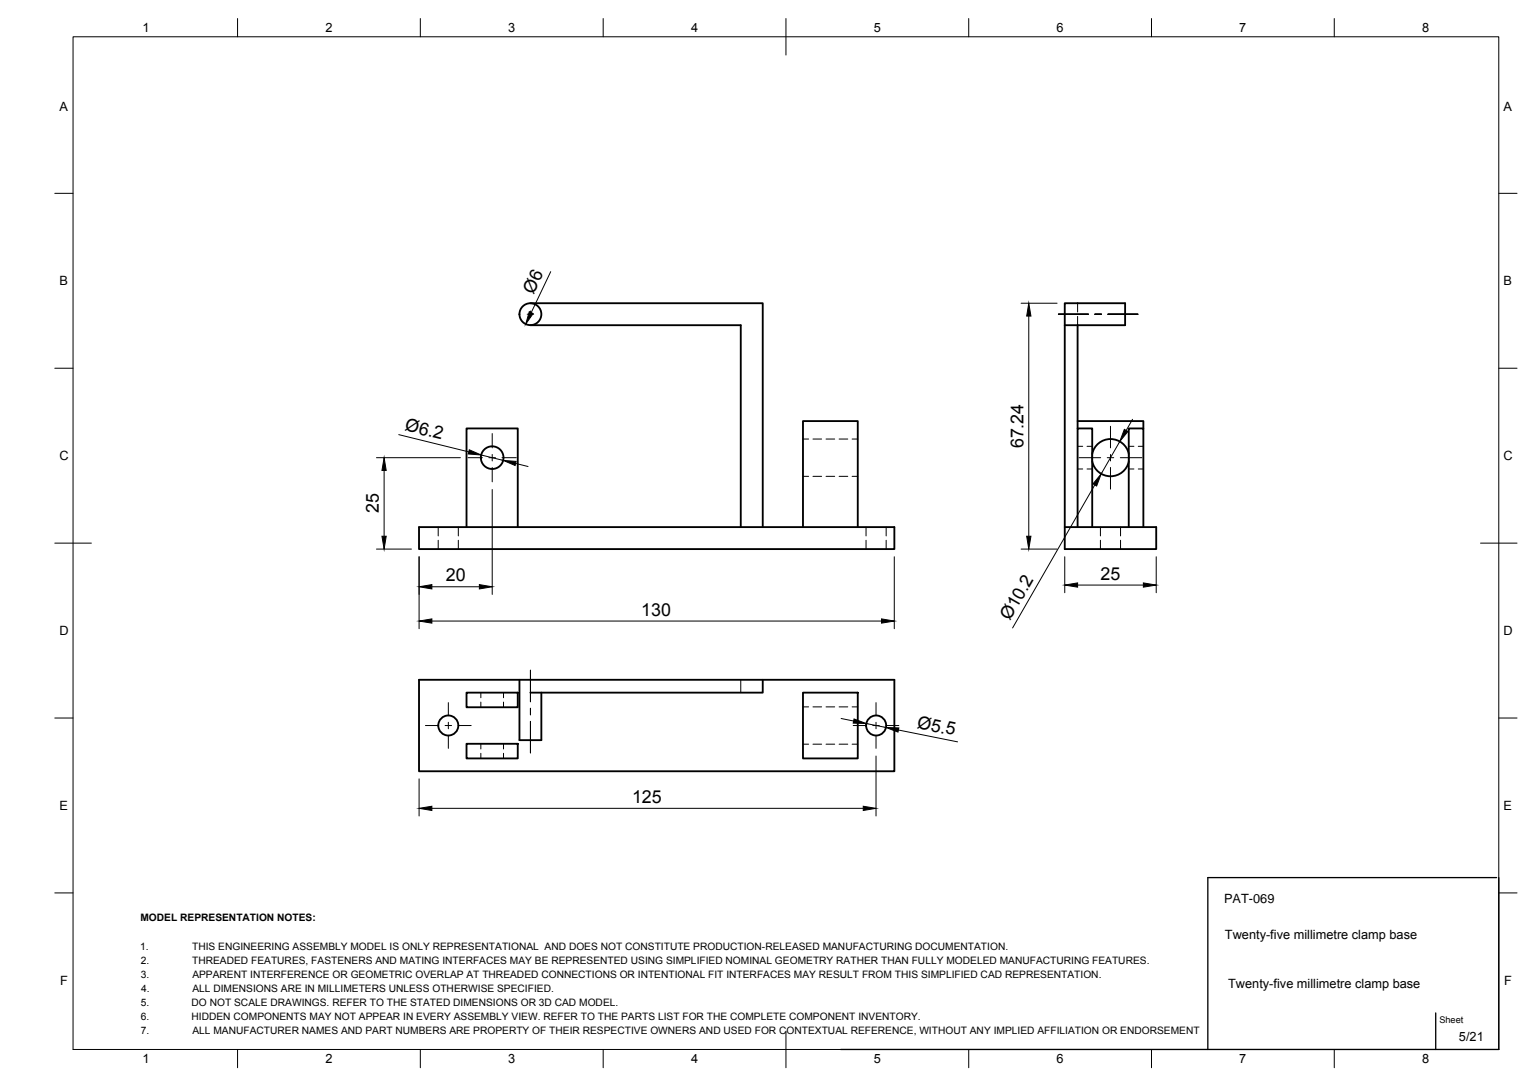
ISO-10303-21;
HEADER;
/* Generated by software containing ST-Developer
 * from STEP Tools, Inc. (www.steptools.com) 
 */

FILE_DESCRIPTION(
/* description */ ('Located fixture plate with toggle clamp'),
/* implementation_level */ '2;1');

FILE_NAME(
/* name */ 'Twenty-five millimetre clamp base.step',
/* time_stamp */ '2026-10-27T21:36:12-07:00',
/* author */ (''),
/* organization */ (''),
/* preprocessor_version */ 'ST-DEVELOPER v20.2',
/* originating_system */ 'Autodesk Translation Framework v15.17.0.0',
/* authorisation */ '');

FILE_SCHEMA (('AUTOMOTIVE_DESIGN { 1 0 10303 214 3 1 1 }'));
ENDSEC;

DATA;
#10=MECHANICAL_DESIGN_GEOMETRIC_PRESENTATION_REPRESENTATION('',(#321),#9285);
#273=SHAPE_REPRESENTATION_RELATIONSHIP('SRR','None',#9396,#297);
#297=ADVANCED_BREP_SHAPE_REPRESENTATION('',(#345),#9258);
#321=STYLED_ITEM('',(#9591),#345);
#345=MANIFOLD_SOLID_BREP('Body1',#5169);
#366=FACE_BOUND('',#977,.T.);
#367=FACE_BOUND('',#978,.T.);
#368=FACE_BOUND('',#979,.T.);
#369=FACE_BOUND('',#980,.T.);
#370=FACE_BOUND('',#981,.T.);
#371=FACE_BOUND('',#987,.T.);
#372=FACE_BOUND('',#989,.T.);
#373=FACE_BOUND('',#995,.T.);
#374=FACE_BOUND('',#1000,.T.);
#375=FACE_BOUND('',#1002,.T.);
#376=FACE_BOUND('',#1007,.T.);
#377=FACE_BOUND('',#1012,.T.);
#378=FACE_BOUND('',#1013,.T.);
#486=PLANE('',#5469);
#487=PLANE('',#5470);
#488=PLANE('',#5471);
#489=PLANE('',#5472);
#490=PLANE('',#5473);
#491=PLANE('',#5474);
#492=PLANE('',#5475);
#493=PLANE('',#5476);
#494=PLANE('',#5486);
#495=PLANE('',#5487);
#496=PLANE('',#5488);
#497=PLANE('',#5489);
#498=PLANE('',#5490);
#499=PLANE('',#5497);
#500=PLANE('',#5498);
#501=PLANE('',#5499);
#502=PLANE('',#5500);
#503=PLANE('',#5501);
#504=PLANE('',#5502);
#505=PLANE('',#5503);
#506=PLANE('',#5504);
#507=PLANE('',#5505);
#508=PLANE('',#5506);
#509=PLANE('',#5507);
#510=PLANE('',#5508);
#511=PLANE('',#5509);
#512=PLANE('',#5510);
#673=FACE_OUTER_BOUND('',#968,.T.);
#674=FACE_OUTER_BOUND('',#969,.T.);
#675=FACE_OUTER_BOUND('',#970,.T.);
#676=FACE_OUTER_BOUND('',#971,.T.);
#677=FACE_OUTER_BOUND('',#972,.T.);
#678=FACE_OUTER_BOUND('',#973,.T.);
#679=FACE_OUTER_BOUND('',#974,.T.);
#680=FACE_OUTER_BOUND('',#975,.T.);
#681=FACE_OUTER_BOUND('',#976,.T.);
#682=FACE_OUTER_BOUND('',#982,.T.);
#683=FACE_OUTER_BOUND('',#983,.T.);
#684=FACE_OUTER_BOUND('',#984,.T.);
#685=FACE_OUTER_BOUND('',#985,.T.);
#686=FACE_OUTER_BOUND('',#986,.T.);
#687=FACE_OUTER_BOUND('',#988,.T.);
#688=FACE_OUTER_BOUND('',#990,.T.);
#689=FACE_OUTER_BOUND('',#991,.T.);
#690=FACE_OUTER_BOUND('',#992,.T.);
#691=FACE_OUTER_BOUND('',#993,.T.);
#692=FACE_OUTER_BOUND('',#994,.T.);
#693=FACE_OUTER_BOUND('',#996,.T.);
#694=FACE_OUTER_BOUND('',#997,.T.);
#695=FACE_OUTER_BOUND('',#998,.T.);
#696=FACE_OUTER_BOUND('',#999,.T.);
#697=FACE_OUTER_BOUND('',#1001,.T.);
#698=FACE_OUTER_BOUND('',#1003,.T.);
#699=FACE_OUTER_BOUND('',#1004,.T.);
#700=FACE_OUTER_BOUND('',#1005,.T.);
#701=FACE_OUTER_BOUND('',#1006,.T.);
#702=FACE_OUTER_BOUND('',#1008,.T.);
#703=FACE_OUTER_BOUND('',#1009,.T.);
#704=FACE_OUTER_BOUND('',#1010,.T.);
#705=FACE_OUTER_BOUND('',#1011,.T.);
#968=EDGE_LOOP('',(#3484,#3485,#3486,#3487,#3488,#3489,#3490,#3491));
#969=EDGE_LOOP('',(#3492));
#970=EDGE_LOOP('',(#3493,#3494,#3495,#3496,#3497,#3498,#3499,#3500,#3501,
#3502,#3503));
#971=EDGE_LOOP('',(#3504,#3505,#3506,#3507));
#972=EDGE_LOOP('',(#3508,#3509,#3510,#3511));
#973=EDGE_LOOP('',(#3512,#3513,#3514,#3515));
#974=EDGE_LOOP('',(#3516,#3517,#3518,#3519));
#975=EDGE_LOOP('',(#3520,#3521,#3522,#3523,#3524,#3525));
#976=EDGE_LOOP('',(#3526,#3527,#3528,#3529,#3530,#3531,#3532,#3533));
#977=EDGE_LOOP('',(#3534,#3535,#3536,#3537));
#978=EDGE_LOOP('',(#3538,#3539,#3540,#3541));
#979=EDGE_LOOP('',(#3542,#3543,#3544,#3545));
#980=EDGE_LOOP('',(#3546));
#981=EDGE_LOOP('',(#3547));
#982=EDGE_LOOP('',(#3548,#3549,#3550,#3551));
#983=EDGE_LOOP('',(#3552,#3553,#3554,#3555));
#984=EDGE_LOOP('',(#3556,#3557,#3558,#3559));
#985=EDGE_LOOP('',(#3560,#3561,#3562,#3563));
#986=EDGE_LOOP('',(#3564,#3565,#3566,#3567));
#987=EDGE_LOOP('',(#3568));
#988=EDGE_LOOP('',(#3569,#3570,#3571,#3572));
#989=EDGE_LOOP('',(#3573));
#990=EDGE_LOOP('',(#3574,#3575,#3576,#3577));
#991=EDGE_LOOP('',(#3578,#3579,#3580,#3581));
#992=EDGE_LOOP('',(#3582,#3583,#3584,#3585));
#993=EDGE_LOOP('',(#3586,#3587,#3588,#3589));
#994=EDGE_LOOP('',(#3590,#3591,#3592,#3593));
#995=EDGE_LOOP('',(#3594));
#996=EDGE_LOOP('',(#3595,#3596,#3597,#3598));
#997=EDGE_LOOP('',(#3599,#3600,#3601,#3602));
#998=EDGE_LOOP('',(#3603,#3604,#3605,#3606));
#999=EDGE_LOOP('',(#3607,#3608,#3609,#3610));
#1000=EDGE_LOOP('',(#3611));
#1001=EDGE_LOOP('',(#3612,#3613,#3614,#3615));
#1002=EDGE_LOOP('',(#3616));
#1003=EDGE_LOOP('',(#3617,#3618,#3619,#3620));
#1004=EDGE_LOOP('',(#3621,#3622,#3623,#3624));
#1005=EDGE_LOOP('',(#3625,#3626,#3627,#3628));
#1006=EDGE_LOOP('',(#3629,#3630,#3631,#3632));
#1007=EDGE_LOOP('',(#3633));
#1008=EDGE_LOOP('',(#3634,#3635,#3636,#3637));
#1009=EDGE_LOOP('',(#3638,#3639,#3640,#3641));
#1010=EDGE_LOOP('',(#3642,#3643,#3644,#3645));
#1011=EDGE_LOOP('',(#3646,#3647,#3648,#3649));
#1012=EDGE_LOOP('',(#3650));
#1013=EDGE_LOOP('',(#3651));
#1383=CIRCLE('',#5465,0.3);
#1384=CIRCLE('',#5466,0.3);
#1385=CIRCLE('',#5467,0.3);
#1386=CIRCLE('',#5468,0.3);
#1387=CIRCLE('',#5477,0.275);
#1388=CIRCLE('',#5478,0.275);
#1389=CIRCLE('',#5480,0.275);
#1390=CIRCLE('',#5482,0.275);
#1391=CIRCLE('',#5484,0.51);
#1392=CIRCLE('',#5485,0.51);
#1393=CIRCLE('',#5492,0.31);
#1394=CIRCLE('',#5493,0.31);
#1395=CIRCLE('',#5495,0.31);
#1396=CIRCLE('',#5496,0.31);
#1581=LINE('',#7581,#1991);
#1582=LINE('',#7585,#1992);
#1583=LINE('',#7589,#1993);
#1584=LINE('',#7595,#1994);
#1585=LINE('',#7597,#1995);
#1586=LINE('',#7599,#1996);
#1587=LINE('',#7601,#1997);
#1588=LINE('',#7603,#1998);
#1589=LINE('',#7605,#1999);
#1590=LINE('',#7607,#2000);
#1591=LINE('',#7609,#2001);
#1592=LINE('',#7610,#2002);
#1593=LINE('',#7613,#2003);
#1594=LINE('',#7614,#2004);
#1595=LINE('',#7617,#2005);
#1596=LINE('',#7618,#2006);
#1597=LINE('',#7621,#2007);
#1598=LINE('',#7622,#2008);
#1599=LINE('',#7625,#2009);
#1600=LINE('',#7626,#2010);
#1601=LINE('',#7628,#2011);
#1602=LINE('',#7631,#2012);
#1603=LINE('',#7633,#2013);
#1604=LINE('',#7634,#2014);
#1605=LINE('',#7637,#2015);
#1606=LINE('',#7639,#2016);
#1607=LINE('',#7641,#2017);
#1608=LINE('',#7642,#2018);
#1609=LINE('',#7645,#2019);
#1610=LINE('',#7647,#2020);
#1611=LINE('',#7649,#2021);
#1612=LINE('',#7650,#2022);
#1613=LINE('',#7653,#2023);
#1614=LINE('',#7655,#2024);
#1615=LINE('',#7657,#2025);
#1616=LINE('',#7658,#2026);
#1617=LINE('',#7666,#2027);
#1618=LINE('',#7670,#2028);
#1619=LINE('',#7675,#2029);
#1620=LINE('',#7679,#2030);
#1621=LINE('',#7681,#2031);
#1622=LINE('',#7682,#2032);
#1623=LINE('',#7685,#2033);
#1624=LINE('',#7686,#2034);
#1625=LINE('',#7689,#2035);
#1626=LINE('',#7690,#2036);
#1627=LINE('',#7692,#2037);
#1628=LINE('',#7698,#2038);
#1629=LINE('',#7704,#2039);
#1630=LINE('',#7708,#2040);
#1631=LINE('',#7710,#2041);
#1632=LINE('',#7711,#2042);
#1633=LINE('',#7714,#2043);
#1634=LINE('',#7715,#2044);
#1635=LINE('',#7718,#2045);
#1636=LINE('',#7719,#2046);
#1637=LINE('',#7721,#2047);
#1638=LINE('',#7725,#2048);
#1639=LINE('',#7727,#2049);
#1640=LINE('',#7728,#2050);
#1641=LINE('',#7731,#2051);
#1642=LINE('',#7732,#2052);
#1643=LINE('',#7735,#2053);
#1644=LINE('',#7736,#2054);
#1645=LINE('',#7738,#2055);
#1646=LINE('',#7742,#2056);
#1647=LINE('',#7743,#2057);
#1648=LINE('',#7746,#2058);
#1649=LINE('',#7747,#2059);
#1650=LINE('',#7749,#2060);
#1991=VECTOR('',#6037,1.);
#1992=VECTOR('',#6040,1.);
#1993=VECTOR('',#6043,0.3);
#1994=VECTOR('',#6052,1.);
#1995=VECTOR('',#6053,1.);
#1996=VECTOR('',#6054,1.);
#1997=VECTOR('',#6055,1.);
#1998=VECTOR('',#6056,1.);
#1999=VECTOR('',#6057,1.);
#2000=VECTOR('',#6058,1.);
#2001=VECTOR('',#6059,1.);
#2002=VECTOR('',#6060,1.);
#2003=VECTOR('',#6063,1.);
#2004=VECTOR('',#6064,1.);
#2005=VECTOR('',#6067,1.);
#2006=VECTOR('',#6068,1.);
#2007=VECTOR('',#6071,1.);
#2008=VECTOR('',#6072,1.);
#2009=VECTOR('',#6075,1.);
#2010=VECTOR('',#6076,1.);
#2011=VECTOR('',#6079,1.);
#2012=VECTOR('',#6082,1.);
#2013=VECTOR('',#6083,1.);
#2014=VECTOR('',#6084,1.);
#2015=VECTOR('',#6085,1.);
#2016=VECTOR('',#6086,1.);
#2017=VECTOR('',#6087,1.);
#2018=VECTOR('',#6088,1.);
#2019=VECTOR('',#6089,1.);
#2020=VECTOR('',#6090,1.);
#2021=VECTOR('',#6091,1.);
#2022=VECTOR('',#6092,1.);
#2023=VECTOR('',#6093,1.);
#2024=VECTOR('',#6094,1.);
#2025=VECTOR('',#6095,1.);
#2026=VECTOR('',#6096,1.);
#2027=VECTOR('',#6105,0.275);
#2028=VECTOR('',#6110,0.275);
#2029=VECTOR('',#6115,0.51);
#2030=VECTOR('',#6120,1.);
#2031=VECTOR('',#6121,1.);
#2032=VECTOR('',#6122,1.);
#2033=VECTOR('',#6125,1.);
#2034=VECTOR('',#6126,1.);
#2035=VECTOR('',#6129,1.);
#2036=VECTOR('',#6130,1.);
#2037=VECTOR('',#6133,1.);
#2038=VECTOR('',#6140,0.31);
#2039=VECTOR('',#6147,0.31);
#2040=VECTOR('',#6152,1.);
#2041=VECTOR('',#6153,1.);
#2042=VECTOR('',#6154,1.);
#2043=VECTOR('',#6157,1.);
#2044=VECTOR('',#6158,1.);
#2045=VECTOR('',#6161,1.);
#2046=VECTOR('',#6162,1.);
#2047=VECTOR('',#6165,1.);
#2048=VECTOR('',#6170,1.);
#2049=VECTOR('',#6171,1.);
#2050=VECTOR('',#6172,1.);
#2051=VECTOR('',#6175,1.);
#2052=VECTOR('',#6176,1.);
#2053=VECTOR('',#6179,1.);
#2054=VECTOR('',#6180,1.);
#2055=VECTOR('',#6183,1.);
#2056=VECTOR('',#6188,1.);
#2057=VECTOR('',#6189,1.);
#2058=VECTOR('',#6192,1.);
#2059=VECTOR('',#6193,1.);
#2060=VECTOR('',#6196,1.);
#2401=VERTEX_POINT('',#7579);
#2402=VERTEX_POINT('',#7580);
#2403=VERTEX_POINT('',#7582);
#2404=VERTEX_POINT('',#7584);
#2405=VERTEX_POINT('',#7586);
#2406=VERTEX_POINT('',#7588);
#2407=VERTEX_POINT('',#7594);
#2408=VERTEX_POINT('',#7596);
#2409=VERTEX_POINT('',#7598);
#2410=VERTEX_POINT('',#7600);
#2411=VERTEX_POINT('',#7602);
#2412=VERTEX_POINT('',#7604);
#2413=VERTEX_POINT('',#7606);
#2414=VERTEX_POINT('',#7608);
#2415=VERTEX_POINT('',#7612);
#2416=VERTEX_POINT('',#7616);
#2417=VERTEX_POINT('',#7620);
#2418=VERTEX_POINT('',#7624);
#2419=VERTEX_POINT('',#7630);
#2420=VERTEX_POINT('',#7632);
#2421=VERTEX_POINT('',#7635);
#2422=VERTEX_POINT('',#7636);
#2423=VERTEX_POINT('',#7638);
#2424=VERTEX_POINT('',#7640);
#2425=VERTEX_POINT('',#7643);
#2426=VERTEX_POINT('',#7644);
#2427=VERTEX_POINT('',#7646);
#2428=VERTEX_POINT('',#7648);
#2429=VERTEX_POINT('',#7651);
#2430=VERTEX_POINT('',#7652);
#2431=VERTEX_POINT('',#7654);
#2432=VERTEX_POINT('',#7656);
#2433=VERTEX_POINT('',#7659);
#2434=VERTEX_POINT('',#7661);
#2435=VERTEX_POINT('',#7664);
#2436=VERTEX_POINT('',#7668);
#2437=VERTEX_POINT('',#7672);
#2438=VERTEX_POINT('',#7674);
#2439=VERTEX_POINT('',#7678);
#2440=VERTEX_POINT('',#7680);
#2441=VERTEX_POINT('',#7684);
#2442=VERTEX_POINT('',#7688);
#2443=VERTEX_POINT('',#7695);
#2444=VERTEX_POINT('',#7697);
#2445=VERTEX_POINT('',#7701);
#2446=VERTEX_POINT('',#7703);
#2447=VERTEX_POINT('',#7707);
#2448=VERTEX_POINT('',#7709);
#2449=VERTEX_POINT('',#7713);
#2450=VERTEX_POINT('',#7717);
#2451=VERTEX_POINT('',#7724);
#2452=VERTEX_POINT('',#7726);
#2453=VERTEX_POINT('',#7730);
#2454=VERTEX_POINT('',#7734);
#2455=VERTEX_POINT('',#7741);
#2456=VERTEX_POINT('',#7745);
#2830=EDGE_CURVE('',#2401,#2402,#1581,.T.);
#2831=EDGE_CURVE('',#2403,#2401,#1383,.T.);
#2832=EDGE_CURVE('',#2403,#2404,#1582,.T.);
#2833=EDGE_CURVE('',#2405,#2404,#1384,.T.);
#2834=EDGE_CURVE('',#2405,#2406,#1583,.T.);
#2835=EDGE_CURVE('',#2406,#2406,#1385,.T.);
#2836=EDGE_CURVE('',#2402,#2405,#1386,.T.);
#2837=EDGE_CURVE('',#2404,#2407,#1584,.T.);
#2838=EDGE_CURVE('',#2407,#2408,#1585,.T.);
#2839=EDGE_CURVE('',#2409,#2408,#1586,.T.);
#2840=EDGE_CURVE('',#2410,#2409,#1587,.T.);
#2841=EDGE_CURVE('',#2410,#2411,#1588,.T.);
#2842=EDGE_CURVE('',#2411,#2412,#1589,.T.);
#2843=EDGE_CURVE('',#2413,#2412,#1590,.T.);
#2844=EDGE_CURVE('',#2413,#2414,#1591,.T.);
#2845=EDGE_CURVE('',#2414,#2402,#1592,.T.);
#2846=EDGE_CURVE('',#2415,#2414,#1593,.T.);
#2847=EDGE_CURVE('',#2401,#2415,#1594,.T.);
#2848=EDGE_CURVE('',#2416,#2403,#1595,.T.);
#2849=EDGE_CURVE('',#2416,#2407,#1596,.T.);
#2850=EDGE_CURVE('',#2417,#2416,#1597,.T.);
#2851=EDGE_CURVE('',#2408,#2417,#1598,.T.);
#2852=EDGE_CURVE('',#2418,#2413,#1599,.T.);
#2853=EDGE_CURVE('',#2415,#2418,#1600,.T.);
#2854=EDGE_CURVE('',#2417,#2418,#1601,.T.);
#2855=EDGE_CURVE('',#2412,#2419,#1602,.T.);
#2856=EDGE_CURVE('',#2419,#2420,#1603,.T.);
#2857=EDGE_CURVE('',#2420,#2409,#1604,.T.);
#2858=EDGE_CURVE('',#2421,#2422,#1605,.T.);
#2859=EDGE_CURVE('',#2422,#2423,#1606,.T.);
#2860=EDGE_CURVE('',#2423,#2424,#1607,.T.);
#2861=EDGE_CURVE('',#2424,#2421,#1608,.T.);
#2862=EDGE_CURVE('',#2425,#2426,#1609,.T.);
#2863=EDGE_CURVE('',#2426,#2427,#1610,.T.);
#2864=EDGE_CURVE('',#2427,#2428,#1611,.T.);
#2865=EDGE_CURVE('',#2428,#2425,#1612,.T.);
#2866=EDGE_CURVE('',#2429,#2430,#1613,.T.);
#2867=EDGE_CURVE('',#2430,#2431,#1614,.T.);
#2868=EDGE_CURVE('',#2431,#2432,#1615,.T.);
#2869=EDGE_CURVE('',#2432,#2429,#1616,.T.);
#2870=EDGE_CURVE('',#2433,#2433,#1387,.T.);
#2871=EDGE_CURVE('',#2434,#2434,#1388,.T.);
#2872=EDGE_CURVE('',#2435,#2435,#1389,.T.);
#2873=EDGE_CURVE('',#2435,#2434,#1617,.T.);
#2874=EDGE_CURVE('',#2436,#2436,#1390,.T.);
#2875=EDGE_CURVE('',#2436,#2433,#1618,.T.);
#2876=EDGE_CURVE('',#2437,#2437,#1391,.T.);
#2877=EDGE_CURVE('',#2437,#2438,#1619,.T.);
#2878=EDGE_CURVE('',#2438,#2438,#1392,.T.);
#2879=EDGE_CURVE('',#2430,#2439,#1620,.T.);
#2880=EDGE_CURVE('',#2439,#2440,#1621,.T.);
#2881=EDGE_CURVE('',#2440,#2431,#1622,.T.);
#2882=EDGE_CURVE('',#2441,#2429,#1623,.T.);
#2883=EDGE_CURVE('',#2439,#2441,#1624,.T.);
#2884=EDGE_CURVE('',#2440,#2442,#1625,.T.);
#2885=EDGE_CURVE('',#2432,#2442,#1626,.T.);
#2886=EDGE_CURVE('',#2442,#2441,#1627,.T.);
#2887=EDGE_CURVE('',#2443,#2443,#1393,.T.);
#2888=EDGE_CURVE('',#2443,#2444,#1628,.T.);
#2889=EDGE_CURVE('',#2444,#2444,#1394,.T.);
#2890=EDGE_CURVE('',#2445,#2445,#1395,.T.);
#2891=EDGE_CURVE('',#2445,#2446,#1629,.T.);
#2892=EDGE_CURVE('',#2446,#2446,#1396,.T.);
#2893=EDGE_CURVE('',#2426,#2447,#1630,.T.);
#2894=EDGE_CURVE('',#2447,#2448,#1631,.T.);
#2895=EDGE_CURVE('',#2448,#2427,#1632,.T.);
#2896=EDGE_CURVE('',#2449,#2425,#1633,.T.);
#2897=EDGE_CURVE('',#2447,#2449,#1634,.T.);
#2898=EDGE_CURVE('',#2448,#2450,#1635,.T.);
#2899=EDGE_CURVE('',#2428,#2450,#1636,.T.);
#2900=EDGE_CURVE('',#2450,#2449,#1637,.T.);
#2901=EDGE_CURVE('',#2422,#2451,#1638,.T.);
#2902=EDGE_CURVE('',#2451,#2452,#1639,.T.);
#2903=EDGE_CURVE('',#2452,#2423,#1640,.T.);
#2904=EDGE_CURVE('',#2453,#2421,#1641,.T.);
#2905=EDGE_CURVE('',#2451,#2453,#1642,.T.);
#2906=EDGE_CURVE('',#2452,#2454,#1643,.T.);
#2907=EDGE_CURVE('',#2424,#2454,#1644,.T.);
#2908=EDGE_CURVE('',#2454,#2453,#1645,.T.);
#2909=EDGE_CURVE('',#2455,#2410,#1646,.T.);
#2910=EDGE_CURVE('',#2455,#2420,#1647,.T.);
#2911=EDGE_CURVE('',#2456,#2455,#1648,.T.);
#2912=EDGE_CURVE('',#2456,#2419,#1649,.T.);
#2913=EDGE_CURVE('',#2411,#2456,#1650,.T.);
#3484=ORIENTED_EDGE('',*,*,#2830,.F.);
#3485=ORIENTED_EDGE('',*,*,#2831,.F.);
#3486=ORIENTED_EDGE('',*,*,#2832,.T.);
#3487=ORIENTED_EDGE('',*,*,#2833,.F.);
#3488=ORIENTED_EDGE('',*,*,#2834,.T.);
#3489=ORIENTED_EDGE('',*,*,#2835,.T.);
#3490=ORIENTED_EDGE('',*,*,#2834,.F.);
#3491=ORIENTED_EDGE('',*,*,#2836,.F.);
#3492=ORIENTED_EDGE('',*,*,#2835,.F.);
#3493=ORIENTED_EDGE('',*,*,#2837,.T.);
#3494=ORIENTED_EDGE('',*,*,#2838,.T.);
#3495=ORIENTED_EDGE('',*,*,#2839,.F.);
#3496=ORIENTED_EDGE('',*,*,#2840,.F.);
#3497=ORIENTED_EDGE('',*,*,#2841,.T.);
#3498=ORIENTED_EDGE('',*,*,#2842,.T.);
#3499=ORIENTED_EDGE('',*,*,#2843,.F.);
#3500=ORIENTED_EDGE('',*,*,#2844,.T.);
#3501=ORIENTED_EDGE('',*,*,#2845,.T.);
#3502=ORIENTED_EDGE('',*,*,#2836,.T.);
#3503=ORIENTED_EDGE('',*,*,#2833,.T.);
#3504=ORIENTED_EDGE('',*,*,#2846,.F.);
#3505=ORIENTED_EDGE('',*,*,#2847,.F.);
#3506=ORIENTED_EDGE('',*,*,#2830,.T.);
#3507=ORIENTED_EDGE('',*,*,#2845,.F.);
#3508=ORIENTED_EDGE('',*,*,#2848,.F.);
#3509=ORIENTED_EDGE('',*,*,#2849,.T.);
#3510=ORIENTED_EDGE('',*,*,#2837,.F.);
#3511=ORIENTED_EDGE('',*,*,#2832,.F.);
#3512=ORIENTED_EDGE('',*,*,#2850,.F.);
#3513=ORIENTED_EDGE('',*,*,#2851,.F.);
#3514=ORIENTED_EDGE('',*,*,#2838,.F.);
#3515=ORIENTED_EDGE('',*,*,#2849,.F.);
#3516=ORIENTED_EDGE('',*,*,#2846,.T.);
#3517=ORIENTED_EDGE('',*,*,#2844,.F.);
#3518=ORIENTED_EDGE('',*,*,#2852,.F.);
#3519=ORIENTED_EDGE('',*,*,#2853,.F.);
#3520=ORIENTED_EDGE('',*,*,#2831,.T.);
#3521=ORIENTED_EDGE('',*,*,#2847,.T.);
#3522=ORIENTED_EDGE('',*,*,#2853,.T.);
#3523=ORIENTED_EDGE('',*,*,#2854,.F.);
#3524=ORIENTED_EDGE('',*,*,#2850,.T.);
#3525=ORIENTED_EDGE('',*,*,#2848,.T.);
#3526=ORIENTED_EDGE('',*,*,#2851,.T.);
#3527=ORIENTED_EDGE('',*,*,#2854,.T.);
#3528=ORIENTED_EDGE('',*,*,#2852,.T.);
#3529=ORIENTED_EDGE('',*,*,#2843,.T.);
#3530=ORIENTED_EDGE('',*,*,#2855,.T.);
#3531=ORIENTED_EDGE('',*,*,#2856,.T.);
#3532=ORIENTED_EDGE('',*,*,#2857,.T.);
#3533=ORIENTED_EDGE('',*,*,#2839,.T.);
#3534=ORIENTED_EDGE('',*,*,#2858,.T.);
#3535=ORIENTED_EDGE('',*,*,#2859,.T.);
#3536=ORIENTED_EDGE('',*,*,#2860,.T.);
#3537=ORIENTED_EDGE('',*,*,#2861,.T.);
#3538=ORIENTED_EDGE('',*,*,#2862,.T.);
#3539=ORIENTED_EDGE('',*,*,#2863,.T.);
#3540=ORIENTED_EDGE('',*,*,#2864,.T.);
#3541=ORIENTED_EDGE('',*,*,#2865,.T.);
#3542=ORIENTED_EDGE('',*,*,#2866,.T.);
#3543=ORIENTED_EDGE('',*,*,#2867,.T.);
#3544=ORIENTED_EDGE('',*,*,#2868,.T.);
#3545=ORIENTED_EDGE('',*,*,#2869,.T.);
#3546=ORIENTED_EDGE('',*,*,#2870,.T.);
#3547=ORIENTED_EDGE('',*,*,#2871,.T.);
#3548=ORIENTED_EDGE('',*,*,#2872,.F.);
#3549=ORIENTED_EDGE('',*,*,#2873,.T.);
#3550=ORIENTED_EDGE('',*,*,#2871,.F.);
#3551=ORIENTED_EDGE('',*,*,#2873,.F.);
#3552=ORIENTED_EDGE('',*,*,#2874,.F.);
#3553=ORIENTED_EDGE('',*,*,#2875,.T.);
#3554=ORIENTED_EDGE('',*,*,#2870,.F.);
#3555=ORIENTED_EDGE('',*,*,#2875,.F.);
#3556=ORIENTED_EDGE('',*,*,#2876,.F.);
#3557=ORIENTED_EDGE('',*,*,#2877,.T.);
#3558=ORIENTED_EDGE('',*,*,#2878,.F.);
#3559=ORIENTED_EDGE('',*,*,#2877,.F.);
#3560=ORIENTED_EDGE('',*,*,#2867,.F.);
#3561=ORIENTED_EDGE('',*,*,#2879,.T.);
#3562=ORIENTED_EDGE('',*,*,#2880,.T.);
#3563=ORIENTED_EDGE('',*,*,#2881,.T.);
#3564=ORIENTED_EDGE('',*,*,#2866,.F.);
#3565=ORIENTED_EDGE('',*,*,#2882,.F.);
#3566=ORIENTED_EDGE('',*,*,#2883,.F.);
#3567=ORIENTED_EDGE('',*,*,#2879,.F.);
#3568=ORIENTED_EDGE('',*,*,#2878,.T.);
#3569=ORIENTED_EDGE('',*,*,#2868,.F.);
#3570=ORIENTED_EDGE('',*,*,#2881,.F.);
#3571=ORIENTED_EDGE('',*,*,#2884,.T.);
#3572=ORIENTED_EDGE('',*,*,#2885,.F.);
#3573=ORIENTED_EDGE('',*,*,#2876,.T.);
#3574=ORIENTED_EDGE('',*,*,#2880,.F.);
#3575=ORIENTED_EDGE('',*,*,#2883,.T.);
#3576=ORIENTED_EDGE('',*,*,#2886,.F.);
#3577=ORIENTED_EDGE('',*,*,#2884,.F.);
#3578=ORIENTED_EDGE('',*,*,#2869,.F.);
#3579=ORIENTED_EDGE('',*,*,#2885,.T.);
#3580=ORIENTED_EDGE('',*,*,#2886,.T.);
#3581=ORIENTED_EDGE('',*,*,#2882,.T.);
#3582=ORIENTED_EDGE('',*,*,#2887,.F.);
#3583=ORIENTED_EDGE('',*,*,#2888,.T.);
#3584=ORIENTED_EDGE('',*,*,#2889,.F.);
#3585=ORIENTED_EDGE('',*,*,#2888,.F.);
#3586=ORIENTED_EDGE('',*,*,#2890,.F.);
#3587=ORIENTED_EDGE('',*,*,#2891,.T.);
#3588=ORIENTED_EDGE('',*,*,#2892,.F.);
#3589=ORIENTED_EDGE('',*,*,#2891,.F.);
#3590=ORIENTED_EDGE('',*,*,#2863,.F.);
#3591=ORIENTED_EDGE('',*,*,#2893,.T.);
#3592=ORIENTED_EDGE('',*,*,#2894,.T.);
#3593=ORIENTED_EDGE('',*,*,#2895,.T.);
#3594=ORIENTED_EDGE('',*,*,#2890,.T.);
#3595=ORIENTED_EDGE('',*,*,#2862,.F.);
#3596=ORIENTED_EDGE('',*,*,#2896,.F.);
#3597=ORIENTED_EDGE('',*,*,#2897,.F.);
#3598=ORIENTED_EDGE('',*,*,#2893,.F.);
#3599=ORIENTED_EDGE('',*,*,#2864,.F.);
#3600=ORIENTED_EDGE('',*,*,#2895,.F.);
#3601=ORIENTED_EDGE('',*,*,#2898,.T.);
#3602=ORIENTED_EDGE('',*,*,#2899,.F.);
#3603=ORIENTED_EDGE('',*,*,#2894,.F.);
#3604=ORIENTED_EDGE('',*,*,#2897,.T.);
#3605=ORIENTED_EDGE('',*,*,#2900,.F.);
#3606=ORIENTED_EDGE('',*,*,#2898,.F.);
#3607=ORIENTED_EDGE('',*,*,#2865,.F.);
#3608=ORIENTED_EDGE('',*,*,#2899,.T.);
#3609=ORIENTED_EDGE('',*,*,#2900,.T.);
#3610=ORIENTED_EDGE('',*,*,#2896,.T.);
#3611=ORIENTED_EDGE('',*,*,#2892,.T.);
#3612=ORIENTED_EDGE('',*,*,#2859,.F.);
#3613=ORIENTED_EDGE('',*,*,#2901,.T.);
#3614=ORIENTED_EDGE('',*,*,#2902,.T.);
#3615=ORIENTED_EDGE('',*,*,#2903,.T.);
#3616=ORIENTED_EDGE('',*,*,#2887,.T.);
#3617=ORIENTED_EDGE('',*,*,#2858,.F.);
#3618=ORIENTED_EDGE('',*,*,#2904,.F.);
#3619=ORIENTED_EDGE('',*,*,#2905,.F.);
#3620=ORIENTED_EDGE('',*,*,#2901,.F.);
#3621=ORIENTED_EDGE('',*,*,#2860,.F.);
#3622=ORIENTED_EDGE('',*,*,#2903,.F.);
#3623=ORIENTED_EDGE('',*,*,#2906,.T.);
#3624=ORIENTED_EDGE('',*,*,#2907,.F.);
#3625=ORIENTED_EDGE('',*,*,#2902,.F.);
#3626=ORIENTED_EDGE('',*,*,#2905,.T.);
#3627=ORIENTED_EDGE('',*,*,#2908,.F.);
#3628=ORIENTED_EDGE('',*,*,#2906,.F.);
#3629=ORIENTED_EDGE('',*,*,#2861,.F.);
#3630=ORIENTED_EDGE('',*,*,#2907,.T.);
#3631=ORIENTED_EDGE('',*,*,#2908,.T.);
#3632=ORIENTED_EDGE('',*,*,#2904,.T.);
#3633=ORIENTED_EDGE('',*,*,#2889,.T.);
#3634=ORIENTED_EDGE('',*,*,#2909,.T.);
#3635=ORIENTED_EDGE('',*,*,#2840,.T.);
#3636=ORIENTED_EDGE('',*,*,#2857,.F.);
#3637=ORIENTED_EDGE('',*,*,#2910,.F.);
#3638=ORIENTED_EDGE('',*,*,#2911,.T.);
#3639=ORIENTED_EDGE('',*,*,#2910,.T.);
#3640=ORIENTED_EDGE('',*,*,#2856,.F.);
#3641=ORIENTED_EDGE('',*,*,#2912,.F.);
#3642=ORIENTED_EDGE('',*,*,#2913,.T.);
#3643=ORIENTED_EDGE('',*,*,#2912,.T.);
#3644=ORIENTED_EDGE('',*,*,#2855,.F.);
#3645=ORIENTED_EDGE('',*,*,#2842,.F.);
#3646=ORIENTED_EDGE('',*,*,#2913,.F.);
#3647=ORIENTED_EDGE('',*,*,#2841,.F.);
#3648=ORIENTED_EDGE('',*,*,#2909,.F.);
#3649=ORIENTED_EDGE('',*,*,#2911,.F.);
#3650=ORIENTED_EDGE('',*,*,#2872,.T.);
#3651=ORIENTED_EDGE('',*,*,#2874,.T.);
#4792=CYLINDRICAL_SURFACE('',#5464,0.3);
#4793=CYLINDRICAL_SURFACE('',#5479,0.275);
#4794=CYLINDRICAL_SURFACE('',#5481,0.275);
#4795=CYLINDRICAL_SURFACE('',#5483,0.51);
#4796=CYLINDRICAL_SURFACE('',#5491,0.31);
#4797=CYLINDRICAL_SURFACE('',#5494,0.31);
#4874=ADVANCED_FACE('',(#673),#4792,.T.);
#4875=ADVANCED_FACE('',(#674),#486,.F.);
#4876=ADVANCED_FACE('',(#675),#487,.T.);
#4877=ADVANCED_FACE('',(#676),#488,.T.);
#4878=ADVANCED_FACE('',(#677),#489,.T.);
#4879=ADVANCED_FACE('',(#678),#490,.T.);
#4880=ADVANCED_FACE('',(#679),#491,.T.);
#4881=ADVANCED_FACE('',(#680),#492,.F.);
#4882=ADVANCED_FACE('',(#681,#366,#367,#368,#369,#370),#493,.T.);
#4883=ADVANCED_FACE('',(#682),#4793,.F.);
#4884=ADVANCED_FACE('',(#683),#4794,.F.);
#4885=ADVANCED_FACE('',(#684),#4795,.F.);
#4886=ADVANCED_FACE('',(#685),#494,.F.);
#4887=ADVANCED_FACE('',(#686,#371),#495,.T.);
#4888=ADVANCED_FACE('',(#687,#372),#496,.T.);
#4889=ADVANCED_FACE('',(#688),#497,.T.);
#4890=ADVANCED_FACE('',(#689),#498,.T.);
#4891=ADVANCED_FACE('',(#690),#4796,.F.);
#4892=ADVANCED_FACE('',(#691),#4797,.F.);
#4893=ADVANCED_FACE('',(#692,#373),#499,.F.);
#4894=ADVANCED_FACE('',(#693),#500,.T.);
#4895=ADVANCED_FACE('',(#694),#501,.T.);
#4896=ADVANCED_FACE('',(#695),#502,.T.);
#4897=ADVANCED_FACE('',(#696,#374),#503,.T.);
#4898=ADVANCED_FACE('',(#697,#375),#504,.F.);
#4899=ADVANCED_FACE('',(#698),#505,.T.);
#4900=ADVANCED_FACE('',(#699),#506,.T.);
#4901=ADVANCED_FACE('',(#700),#507,.T.);
#4902=ADVANCED_FACE('',(#701,#376),#508,.T.);
#4903=ADVANCED_FACE('',(#702),#509,.T.);
#4904=ADVANCED_FACE('',(#703),#510,.T.);
#4905=ADVANCED_FACE('',(#704),#511,.T.);
#4906=ADVANCED_FACE('',(#705,#377,#378),#512,.F.);
#5169=CLOSED_SHELL('',(#4874,#4875,#4876,#4877,#4878,#4879,#4880,#4881,
#4882,#4883,#4884,#4885,#4886,#4887,#4888,#4889,#4890,#4891,#4892,#4893,
#4894,#4895,#4896,#4897,#4898,#4899,#4900,#4901,#4902,#4903,#4904,#4905,
#4906));
#5463=AXIS2_PLACEMENT_3D('',#7577,#6033,#6034);
#5464=AXIS2_PLACEMENT_3D('',#7578,#6035,#6036);
#5465=AXIS2_PLACEMENT_3D('',#7583,#6038,#6039);
#5466=AXIS2_PLACEMENT_3D('',#7587,#6041,#6042);
#5467=AXIS2_PLACEMENT_3D('',#7590,#6044,#6045);
#5468=AXIS2_PLACEMENT_3D('',#7591,#6046,#6047);
#5469=AXIS2_PLACEMENT_3D('',#7592,#6048,#6049);
#5470=AXIS2_PLACEMENT_3D('',#7593,#6050,#6051);
#5471=AXIS2_PLACEMENT_3D('',#7611,#6061,#6062);
#5472=AXIS2_PLACEMENT_3D('',#7615,#6065,#6066);
#5473=AXIS2_PLACEMENT_3D('',#7619,#6069,#6070);
#5474=AXIS2_PLACEMENT_3D('',#7623,#6073,#6074);
#5475=AXIS2_PLACEMENT_3D('',#7627,#6077,#6078);
#5476=AXIS2_PLACEMENT_3D('',#7629,#6080,#6081);
#5477=AXIS2_PLACEMENT_3D('',#7660,#6097,#6098);
#5478=AXIS2_PLACEMENT_3D('',#7662,#6099,#6100);
#5479=AXIS2_PLACEMENT_3D('',#7663,#6101,#6102);
#5480=AXIS2_PLACEMENT_3D('',#7665,#6103,#6104);
#5481=AXIS2_PLACEMENT_3D('',#7667,#6106,#6107);
#5482=AXIS2_PLACEMENT_3D('',#7669,#6108,#6109);
#5483=AXIS2_PLACEMENT_3D('',#7671,#6111,#6112);
#5484=AXIS2_PLACEMENT_3D('',#7673,#6113,#6114);
#5485=AXIS2_PLACEMENT_3D('',#7676,#6116,#6117);
#5486=AXIS2_PLACEMENT_3D('',#7677,#6118,#6119);
#5487=AXIS2_PLACEMENT_3D('',#7683,#6123,#6124);
#5488=AXIS2_PLACEMENT_3D('',#7687,#6127,#6128);
#5489=AXIS2_PLACEMENT_3D('',#7691,#6131,#6132);
#5490=AXIS2_PLACEMENT_3D('',#7693,#6134,#6135);
#5491=AXIS2_PLACEMENT_3D('',#7694,#6136,#6137);
#5492=AXIS2_PLACEMENT_3D('',#7696,#6138,#6139);
#5493=AXIS2_PLACEMENT_3D('',#7699,#6141,#6142);
#5494=AXIS2_PLACEMENT_3D('',#7700,#6143,#6144);
#5495=AXIS2_PLACEMENT_3D('',#7702,#6145,#6146);
#5496=AXIS2_PLACEMENT_3D('',#7705,#6148,#6149);
#5497=AXIS2_PLACEMENT_3D('',#7706,#6150,#6151);
#5498=AXIS2_PLACEMENT_3D('',#7712,#6155,#6156);
#5499=AXIS2_PLACEMENT_3D('',#7716,#6159,#6160);
#5500=AXIS2_PLACEMENT_3D('',#7720,#6163,#6164);
#5501=AXIS2_PLACEMENT_3D('',#7722,#6166,#6167);
#5502=AXIS2_PLACEMENT_3D('',#7723,#6168,#6169);
#5503=AXIS2_PLACEMENT_3D('',#7729,#6173,#6174);
#5504=AXIS2_PLACEMENT_3D('',#7733,#6177,#6178);
#5505=AXIS2_PLACEMENT_3D('',#7737,#6181,#6182);
#5506=AXIS2_PLACEMENT_3D('',#7739,#6184,#6185);
#5507=AXIS2_PLACEMENT_3D('',#7740,#6186,#6187);
#5508=AXIS2_PLACEMENT_3D('',#7744,#6190,#6191);
#5509=AXIS2_PLACEMENT_3D('',#7748,#6194,#6195);
#5510=AXIS2_PLACEMENT_3D('',#7750,#6197,#6198);
#6033=DIRECTION('axis',(0.,0.,1.));
#6034=DIRECTION('refdir',(1.,0.,0.));
#6035=DIRECTION('center_axis',(0.,1.,0.));
#6036=DIRECTION('ref_axis',(1.,0.,0.));
#6037=DIRECTION('',(0.,1.,0.));
#6038=DIRECTION('center_axis',(0.,1.,0.));
#6039=DIRECTION('ref_axis',(1.,0.,0.));
#6040=DIRECTION('',(0.,1.,0.));
#6041=DIRECTION('center_axis',(0.,1.,0.));
#6042=DIRECTION('ref_axis',(1.,0.,0.));
#6043=DIRECTION('',(0.,-1.,0.));
#6044=DIRECTION('center_axis',(0.,1.,0.));
#6045=DIRECTION('ref_axis',(1.,0.,0.));
#6046=DIRECTION('center_axis',(0.,1.,0.));
#6047=DIRECTION('ref_axis',(1.,0.,0.));
#6048=DIRECTION('center_axis',(0.,1.,0.));
#6049=DIRECTION('ref_axis',(1.,0.,0.));
#6050=DIRECTION('center_axis',(0.,1.,0.));
#6051=DIRECTION('ref_axis',(-1.,0.,0.));
#6052=DIRECTION('',(1.,0.,0.));
#6053=DIRECTION('',(0.,0.,-1.));
#6054=DIRECTION('',(-1.,0.,0.));
#6055=DIRECTION('',(0.,0.,1.));
#6056=DIRECTION('',(-1.,0.,0.));
#6057=DIRECTION('',(0.,0.,1.));
#6058=DIRECTION('',(-1.,0.,0.));
#6059=DIRECTION('',(0.,0.,1.));
#6060=DIRECTION('',(-1.,0.,0.));
#6061=DIRECTION('center_axis',(0.,0.,-1.));
#6062=DIRECTION('ref_axis',(-1.,0.,0.));
#6063=DIRECTION('',(0.,1.,0.));
#6064=DIRECTION('',(1.,0.,0.));
#6065=DIRECTION('center_axis',(0.,0.,1.));
#6066=DIRECTION('ref_axis',(1.,0.,0.));
#6067=DIRECTION('',(-1.,0.,0.));
#6068=DIRECTION('',(0.,1.,0.));
#6069=DIRECTION('center_axis',(1.,0.,0.));
#6070=DIRECTION('ref_axis',(0.,0.,-1.));
#6071=DIRECTION('',(0.,0.,1.));
#6072=DIRECTION('',(0.,-1.,0.));
#6073=DIRECTION('center_axis',(-1.,0.,0.));
#6074=DIRECTION('ref_axis',(0.,0.,1.));
#6075=DIRECTION('',(0.,1.,0.));
#6076=DIRECTION('',(0.,0.,-1.));
#6077=DIRECTION('center_axis',(0.,1.,0.));
#6078=DIRECTION('ref_axis',(1.,0.,0.));
#6079=DIRECTION('',(-1.,0.,0.));
#6080=DIRECTION('center_axis',(0.,0.,1.));
#6081=DIRECTION('ref_axis',(1.,0.,0.));
#6082=DIRECTION('',(0.,-1.,0.));
#6083=DIRECTION('',(1.,0.,0.));
#6084=DIRECTION('',(0.,1.,0.));
#6085=DIRECTION('',(0.,-1.,0.));
#6086=DIRECTION('',(-1.,0.,0.));
#6087=DIRECTION('',(0.,1.,0.));
#6088=DIRECTION('',(1.,0.,0.));
#6089=DIRECTION('',(0.,-1.,0.));
#6090=DIRECTION('',(-1.,0.,0.));
#6091=DIRECTION('',(0.,1.,0.));
#6092=DIRECTION('',(1.,0.,0.));
#6093=DIRECTION('',(0.,-1.,0.));
#6094=DIRECTION('',(-1.,0.,0.));
#6095=DIRECTION('',(0.,1.,0.));
#6096=DIRECTION('',(1.,0.,0.));
#6097=DIRECTION('center_axis',(0.,0.,-1.));
#6098=DIRECTION('ref_axis',(1.,0.,0.));
#6099=DIRECTION('center_axis',(0.,0.,-1.));
#6100=DIRECTION('ref_axis',(1.,0.,0.));
#6101=DIRECTION('center_axis',(0.,0.,1.));
#6102=DIRECTION('ref_axis',(1.,0.,0.));
#6103=DIRECTION('center_axis',(0.,0.,1.));
#6104=DIRECTION('ref_axis',(1.,0.,0.));
#6105=DIRECTION('',(0.,0.,1.));
#6106=DIRECTION('center_axis',(0.,0.,1.));
#6107=DIRECTION('ref_axis',(1.,0.,0.));
#6108=DIRECTION('center_axis',(0.,0.,1.));
#6109=DIRECTION('ref_axis',(1.,0.,0.));
#6110=DIRECTION('',(0.,0.,1.));
#6111=DIRECTION('center_axis',(1.,0.,0.));
#6112=DIRECTION('ref_axis',(0.,0.,-1.));
#6113=DIRECTION('center_axis',(1.,0.,0.));
#6114=DIRECTION('ref_axis',(0.,0.,-1.));
#6115=DIRECTION('',(1.,0.,0.));
#6116=DIRECTION('center_axis',(-1.,0.,0.));
#6117=DIRECTION('ref_axis',(0.,0.,-1.));
#6118=DIRECTION('center_axis',(0.,1.,0.));
#6119=DIRECTION('ref_axis',(1.,0.,0.));
#6120=DIRECTION('',(0.,0.,1.));
#6121=DIRECTION('',(-1.,0.,0.));
#6122=DIRECTION('',(0.,0.,-1.));
#6123=DIRECTION('center_axis',(1.,0.,0.));
#6124=DIRECTION('ref_axis',(0.,0.,-1.));
#6125=DIRECTION('',(0.,0.,-1.));
#6126=DIRECTION('',(0.,1.,0.));
#6127=DIRECTION('center_axis',(-1.,0.,0.));
#6128=DIRECTION('ref_axis',(0.,0.,1.));
#6129=DIRECTION('',(0.,1.,0.));
#6130=DIRECTION('',(0.,0.,1.));
#6131=DIRECTION('center_axis',(0.,0.,1.));
#6132=DIRECTION('ref_axis',(1.,0.,0.));
#6133=DIRECTION('',(1.,0.,0.));
#6134=DIRECTION('center_axis',(0.,1.,0.));
#6135=DIRECTION('ref_axis',(0.,0.,1.));
#6136=DIRECTION('center_axis',(0.,1.,0.));
#6137=DIRECTION('ref_axis',(1.,0.,0.));
#6138=DIRECTION('center_axis',(0.,1.,0.));
#6139=DIRECTION('ref_axis',(1.,0.,0.));
#6140=DIRECTION('',(0.,1.,0.));
#6141=DIRECTION('center_axis',(0.,-1.,0.));
#6142=DIRECTION('ref_axis',(1.,0.,0.));
#6143=DIRECTION('center_axis',(0.,1.,0.));
#6144=DIRECTION('ref_axis',(1.,0.,0.));
#6145=DIRECTION('center_axis',(0.,1.,0.));
#6146=DIRECTION('ref_axis',(1.,0.,0.));
#6147=DIRECTION('',(0.,1.,0.));
#6148=DIRECTION('center_axis',(0.,-1.,0.));
#6149=DIRECTION('ref_axis',(1.,0.,0.));
#6150=DIRECTION('center_axis',(0.,1.,0.));
#6151=DIRECTION('ref_axis',(1.,0.,0.));
#6152=DIRECTION('',(0.,0.,1.));
#6153=DIRECTION('',(-1.,0.,0.));
#6154=DIRECTION('',(0.,0.,-1.));
#6155=DIRECTION('center_axis',(1.,0.,0.));
#6156=DIRECTION('ref_axis',(0.,0.,-1.));
#6157=DIRECTION('',(0.,0.,-1.));
#6158=DIRECTION('',(0.,1.,0.));
#6159=DIRECTION('center_axis',(-1.,0.,0.));
#6160=DIRECTION('ref_axis',(0.,0.,1.));
#6161=DIRECTION('',(0.,1.,0.));
#6162=DIRECTION('',(0.,0.,1.));
#6163=DIRECTION('center_axis',(0.,0.,1.));
#6164=DIRECTION('ref_axis',(1.,0.,0.));
#6165=DIRECTION('',(1.,0.,0.));
#6166=DIRECTION('center_axis',(0.,1.,0.));
#6167=DIRECTION('ref_axis',(0.,0.,1.));
#6168=DIRECTION('center_axis',(0.,1.,0.));
#6169=DIRECTION('ref_axis',(1.,0.,0.));
#6170=DIRECTION('',(0.,0.,1.));
#6171=DIRECTION('',(-1.,0.,0.));
#6172=DIRECTION('',(0.,0.,-1.));
#6173=DIRECTION('center_axis',(1.,0.,0.));
#6174=DIRECTION('ref_axis',(0.,0.,-1.));
#6175=DIRECTION('',(0.,0.,-1.));
#6176=DIRECTION('',(0.,1.,0.));
#6177=DIRECTION('center_axis',(-1.,0.,0.));
#6178=DIRECTION('ref_axis',(0.,0.,1.));
#6179=DIRECTION('',(0.,1.,0.));
#6180=DIRECTION('',(0.,0.,1.));
#6181=DIRECTION('center_axis',(0.,0.,1.));
#6182=DIRECTION('ref_axis',(1.,0.,0.));
#6183=DIRECTION('',(1.,0.,0.));
#6184=DIRECTION('center_axis',(0.,1.,0.));
#6185=DIRECTION('ref_axis',(0.,0.,1.));
#6186=DIRECTION('center_axis',(1.,0.,0.));
#6187=DIRECTION('ref_axis',(0.,1.,0.));
#6188=DIRECTION('',(0.,1.,0.));
#6189=DIRECTION('',(0.,0.,1.));
#6190=DIRECTION('center_axis',(0.,-1.,0.));
#6191=DIRECTION('ref_axis',(1.,0.,0.));
#6192=DIRECTION('',(1.,0.,0.));
#6193=DIRECTION('',(0.,0.,1.));
#6194=DIRECTION('center_axis',(-1.,0.,0.));
#6195=DIRECTION('ref_axis',(0.,-1.,0.));
#6196=DIRECTION('',(0.,-1.,0.));
#6197=DIRECTION('center_axis',(0.,0.,1.));
#6198=DIRECTION('ref_axis',(1.,0.,0.));
#7577=CARTESIAN_POINT('',(0.,0.,0.));
#7578=CARTESIAN_POINT('Origin',(1.04595925965485,-0.4,6.42376977244362));
#7579=CARTESIAN_POINT('',(1.04595925965485,0.9,6.12376977244362));
#7580=CARTESIAN_POINT('',(1.04595925965485,1.25,6.12376977244362));
#7581=CARTESIAN_POINT('',(1.04595925965485,0.9,6.12376977244362));
#7582=CARTESIAN_POINT('',(1.04595925965485,0.9,6.72376977244362));
#7583=CARTESIAN_POINT('Origin',(1.04595925965485,0.9,6.42376977244362));
#7584=CARTESIAN_POINT('',(1.04595925965485,1.25,6.72376977244362));
#7585=CARTESIAN_POINT('',(1.04595925965485,0.9,6.72376977244362));
#7586=CARTESIAN_POINT('',(0.745959259654855,1.25,6.42376977244362));
#7587=CARTESIAN_POINT('Origin',(1.04595925965485,1.25,6.42376977244362));
#7588=CARTESIAN_POINT('',(0.745959259654855,-0.4,6.42376977244362));
#7589=CARTESIAN_POINT('',(0.745959259654855,-0.4,6.42376977244362));
#7590=CARTESIAN_POINT('Origin',(1.04595925965485,-0.4,6.42376977244362));
#7591=CARTESIAN_POINT('Origin',(1.04595925965485,1.25,6.42376977244362));
#7592=CARTESIAN_POINT('Origin',(1.04595925965485,-0.4,6.42376977244362));
#7593=CARTESIAN_POINT('Origin',(11.,1.25,0.));
#7594=CARTESIAN_POINT('',(7.4,1.25,6.72376977244362));
#7595=CARTESIAN_POINT('',(7.4,1.25,6.72376977244362));
#7596=CARTESIAN_POINT('',(7.4,1.25,0.6));
#7597=CARTESIAN_POINT('',(7.4,1.25,6.12376977244362));
#7598=CARTESIAN_POINT('',(11.,1.25,0.6));
#7599=CARTESIAN_POINT('',(11.,1.25,0.6));
#7600=CARTESIAN_POINT('',(11.,1.25,0.));
#7601=CARTESIAN_POINT('',(11.,1.25,0.));
#7602=CARTESIAN_POINT('',(-2.,1.25,0.));
#7603=CARTESIAN_POINT('',(11.,1.25,0.));
#7604=CARTESIAN_POINT('',(-2.,1.25,0.6));
#7605=CARTESIAN_POINT('',(-2.,1.25,0.));
#7606=CARTESIAN_POINT('',(6.8,1.25,0.6));
#7607=CARTESIAN_POINT('',(11.,1.25,0.6));
#7608=CARTESIAN_POINT('',(6.8,1.25,6.12376977244362));
#7609=CARTESIAN_POINT('',(6.8,1.25,6.42376977244362));
#7610=CARTESIAN_POINT('',(1.04595925965485,1.25,6.12376977244362));
#7611=CARTESIAN_POINT('Origin',(7.4,0.9,6.12376977244362));
#7612=CARTESIAN_POINT('',(6.8,0.9,6.12376977244362));
#7613=CARTESIAN_POINT('',(6.8,0.9,6.12376977244362));
#7614=CARTESIAN_POINT('',(1.04595925965485,0.9,6.12376977244362));
#7615=CARTESIAN_POINT('Origin',(1.04595925965485,0.9,6.72376977244362));
#7616=CARTESIAN_POINT('',(7.4,0.9,6.72376977244362));
#7617=CARTESIAN_POINT('',(7.4,0.9,6.72376977244362));
#7618=CARTESIAN_POINT('',(7.4,0.9,6.72376977244362));
#7619=CARTESIAN_POINT('Origin',(7.4,0.9,6.42376977244362));
#7620=CARTESIAN_POINT('',(7.4,0.9,0.6));
#7621=CARTESIAN_POINT('',(7.4,0.9,6.12376977244362));
#7622=CARTESIAN_POINT('',(7.4,0.45,0.6));
#7623=CARTESIAN_POINT('Origin',(6.8,0.9,0.5));
#7624=CARTESIAN_POINT('',(6.8,0.9,0.6));
#7625=CARTESIAN_POINT('',(6.8,0.45,0.6));
#7626=CARTESIAN_POINT('',(6.8,0.9,6.42376977244362));
#7627=CARTESIAN_POINT('Origin',(7.1,0.9,3.46188488622181));
#7628=CARTESIAN_POINT('',(5.8,0.9,0.6));
#7629=CARTESIAN_POINT('Origin',(4.5,0.,0.6));
#7630=CARTESIAN_POINT('',(-2.,-1.25,0.6));
#7631=CARTESIAN_POINT('',(-2.,1.25,0.6));
#7632=CARTESIAN_POINT('',(11.,-1.25,0.6));
#7633=CARTESIAN_POINT('',(-2.,-1.25,0.6));
#7634=CARTESIAN_POINT('',(11.,-1.25,0.6));
#7635=CARTESIAN_POINT('',(0.7,-0.5,0.6));
#7636=CARTESIAN_POINT('',(0.7,-0.9,0.6));
#7637=CARTESIAN_POINT('',(0.7,-0.45,0.6));
#7638=CARTESIAN_POINT('',(-0.7,-0.9,0.6));
#7639=CARTESIAN_POINT('',(2.25,-0.9,0.6));
#7640=CARTESIAN_POINT('',(-0.7,-0.5,0.6));
#7641=CARTESIAN_POINT('',(-0.7,-0.45,0.6));
#7642=CARTESIAN_POINT('',(2.25,-0.5,0.6));
#7643=CARTESIAN_POINT('',(0.7,0.9,0.6));
#7644=CARTESIAN_POINT('',(0.7,0.5,0.6));
#7645=CARTESIAN_POINT('',(0.7,0.25,0.6));
#7646=CARTESIAN_POINT('',(-0.7,0.5,0.6));
#7647=CARTESIAN_POINT('',(2.25,0.5,0.6));
#7648=CARTESIAN_POINT('',(-0.7,0.9,0.6));
#7649=CARTESIAN_POINT('',(-0.7,0.25,0.6));
#7650=CARTESIAN_POINT('',(2.25,0.9,0.6));
#7651=CARTESIAN_POINT('',(10.,0.9,0.6));
#7652=CARTESIAN_POINT('',(10.,-0.9,0.6));
#7653=CARTESIAN_POINT('',(10.,-0.45,0.6));
#7654=CARTESIAN_POINT('',(8.5,-0.9,0.6));
#7655=CARTESIAN_POINT('',(6.875,-0.9,0.6));
#7656=CARTESIAN_POINT('',(8.5,0.9,0.6));
#7657=CARTESIAN_POINT('',(8.5,-0.45,0.6));
#7658=CARTESIAN_POINT('',(6.875,0.9,0.6));
#7659=CARTESIAN_POINT('',(10.225,3.36777869765523E-17,0.6));
#7660=CARTESIAN_POINT('Origin',(10.5,0.,0.6));
#7661=CARTESIAN_POINT('',(-1.475,3.36777869765522E-17,0.6));
#7662=CARTESIAN_POINT('Origin',(-1.2,0.,0.6));
#7663=CARTESIAN_POINT('Origin',(-1.2,0.,-0.1));
#7664=CARTESIAN_POINT('',(-1.475,-3.36777869765522E-17,0.));
#7665=CARTESIAN_POINT('Origin',(-1.2,0.,0.));
#7666=CARTESIAN_POINT('',(-1.475,-3.36777869765522E-17,-0.1));
#7667=CARTESIAN_POINT('Origin',(10.5,0.,-0.1));
#7668=CARTESIAN_POINT('',(10.225,-3.36777869765523E-17,0.));
#7669=CARTESIAN_POINT('Origin',(10.5,0.,0.));
#7670=CARTESIAN_POINT('',(10.225,-3.36777869765523E-17,-0.1));
#7671=CARTESIAN_POINT('Origin',(8.4,0.,2.5));
#7672=CARTESIAN_POINT('',(8.5,-6.2456986756515E-17,3.01));
#7673=CARTESIAN_POINT('Origin',(8.5,0.,2.5));
#7674=CARTESIAN_POINT('',(10.,6.2456986756515E-17,3.01));
#7675=CARTESIAN_POINT('',(8.4,-6.2456986756515E-17,3.01));
#7676=CARTESIAN_POINT('Origin',(10.,0.,2.5));
#7677=CARTESIAN_POINT('Origin',(9.25,-0.9,2.));
#7678=CARTESIAN_POINT('',(10.,-0.9,3.5));
#7679=CARTESIAN_POINT('',(10.,-0.9,0.5));
#7680=CARTESIAN_POINT('',(8.5,-0.9,3.5));
#7681=CARTESIAN_POINT('',(10.,-0.9,3.5));
#7682=CARTESIAN_POINT('',(8.5,-0.9,3.5));
#7683=CARTESIAN_POINT('Origin',(10.,-0.9,3.5));
#7684=CARTESIAN_POINT('',(10.,0.9,3.5));
#7685=CARTESIAN_POINT('',(10.,0.9,0.5));
#7686=CARTESIAN_POINT('',(10.,-0.9,3.5));
#7687=CARTESIAN_POINT('Origin',(8.5,-0.9,0.5));
#7688=CARTESIAN_POINT('',(8.5,0.9,3.5));
#7689=CARTESIAN_POINT('',(8.5,-0.9,3.5));
#7690=CARTESIAN_POINT('',(8.5,0.9,3.5));
#7691=CARTESIAN_POINT('Origin',(8.5,-0.9,3.5));
#7692=CARTESIAN_POINT('',(10.,0.9,3.5));
#7693=CARTESIAN_POINT('Origin',(9.25,0.9,2.));
#7694=CARTESIAN_POINT('Origin',(0.,-1.,2.5));
#7695=CARTESIAN_POINT('',(-0.31,-0.9,2.5));
#7696=CARTESIAN_POINT('Origin',(0.,-0.9,2.5));
#7697=CARTESIAN_POINT('',(-0.31,-0.5,2.5));
#7698=CARTESIAN_POINT('',(-0.31,-1.,2.5));
#7699=CARTESIAN_POINT('Origin',(0.,-0.5,2.5));
#7700=CARTESIAN_POINT('Origin',(0.,-1.,2.5));
#7701=CARTESIAN_POINT('',(-0.31,0.5,2.5));
#7702=CARTESIAN_POINT('Origin',(0.,0.5,2.5));
#7703=CARTESIAN_POINT('',(-0.31,0.9,2.5));
#7704=CARTESIAN_POINT('',(-0.31,-1.,2.5));
#7705=CARTESIAN_POINT('Origin',(0.,0.9,2.5));
#7706=CARTESIAN_POINT('Origin',(0.,0.5,1.9));
#7707=CARTESIAN_POINT('',(0.7,0.5,3.3));
#7708=CARTESIAN_POINT('',(0.7,0.5,0.5));
#7709=CARTESIAN_POINT('',(-0.7,0.5,3.3));
#7710=CARTESIAN_POINT('',(0.7,0.5,3.3));
#7711=CARTESIAN_POINT('',(-0.7,0.5,3.3));
#7712=CARTESIAN_POINT('Origin',(0.7,0.5,3.3));
#7713=CARTESIAN_POINT('',(0.7,0.9,3.3));
#7714=CARTESIAN_POINT('',(0.7,0.9,0.5));
#7715=CARTESIAN_POINT('',(0.7,0.5,3.3));
#7716=CARTESIAN_POINT('Origin',(-0.7,0.5,0.5));
#7717=CARTESIAN_POINT('',(-0.7,0.9,3.3));
#7718=CARTESIAN_POINT('',(-0.7,0.5,3.3));
#7719=CARTESIAN_POINT('',(-0.7,0.9,3.3));
#7720=CARTESIAN_POINT('Origin',(-0.7,0.5,3.3));
#7721=CARTESIAN_POINT('',(0.7,0.9,3.3));
#7722=CARTESIAN_POINT('Origin',(0.,0.9,1.9));
#7723=CARTESIAN_POINT('Origin',(0.,-0.9,1.9));
#7724=CARTESIAN_POINT('',(0.7,-0.9,3.3));
#7725=CARTESIAN_POINT('',(0.7,-0.9,0.5));
#7726=CARTESIAN_POINT('',(-0.7,-0.9,3.3));
#7727=CARTESIAN_POINT('',(0.7,-0.9,3.3));
#7728=CARTESIAN_POINT('',(-0.7,-0.9,3.3));
#7729=CARTESIAN_POINT('Origin',(0.7,-0.9,3.3));
#7730=CARTESIAN_POINT('',(0.7,-0.5,3.3));
#7731=CARTESIAN_POINT('',(0.7,-0.5,0.5));
#7732=CARTESIAN_POINT('',(0.7,-0.9,3.3));
#7733=CARTESIAN_POINT('Origin',(-0.7,-0.9,0.5));
#7734=CARTESIAN_POINT('',(-0.7,-0.5,3.3));
#7735=CARTESIAN_POINT('',(-0.7,-0.9,3.3));
#7736=CARTESIAN_POINT('',(-0.7,-0.5,3.3));
#7737=CARTESIAN_POINT('Origin',(-0.7,-0.9,3.3));
#7738=CARTESIAN_POINT('',(0.7,-0.5,3.3));
#7739=CARTESIAN_POINT('Origin',(0.,-0.5,1.9));
#7740=CARTESIAN_POINT('Origin',(11.,-1.25,0.));
#7741=CARTESIAN_POINT('',(11.,-1.25,0.));
#7742=CARTESIAN_POINT('',(11.,-1.25,0.));
#7743=CARTESIAN_POINT('',(11.,-1.25,0.));
#7744=CARTESIAN_POINT('Origin',(-2.,-1.25,0.));
#7745=CARTESIAN_POINT('',(-2.,-1.25,0.));
#7746=CARTESIAN_POINT('',(-2.,-1.25,0.));
#7747=CARTESIAN_POINT('',(-2.,-1.25,0.));
#7748=CARTESIAN_POINT('Origin',(-2.,1.25,0.));
#7749=CARTESIAN_POINT('',(-2.,1.25,0.));
#7750=CARTESIAN_POINT('Origin',(4.5,0.,0.));
#9228=UNCERTAINTY_MEASURE_WITH_UNIT(LENGTH_MEASURE(0.001),#9286,
'DISTANCE_ACCURACY_VALUE',
'Maximum model space distance between geometric entities at asserted c
onnectivities');
#9255=UNCERTAINTY_MEASURE_WITH_UNIT(LENGTH_MEASURE(0.001),#9286,
'DISTANCE_ACCURACY_VALUE',
'Maximum model space distance between geometric entities at asserted c
onnectivities');
#9258=(
GEOMETRIC_REPRESENTATION_CONTEXT(3)
GLOBAL_UNCERTAINTY_ASSIGNED_CONTEXT((#9228))
GLOBAL_UNIT_ASSIGNED_CONTEXT((#9286,#9288,#9289))
REPRESENTATION_CONTEXT('','3D')
);
#9285=(
GEOMETRIC_REPRESENTATION_CONTEXT(3)
GLOBAL_UNCERTAINTY_ASSIGNED_CONTEXT((#9255))
GLOBAL_UNIT_ASSIGNED_CONTEXT((#9286,#9288,#9289))
REPRESENTATION_CONTEXT('','3D')
);
#9286=(
LENGTH_UNIT()
NAMED_UNIT(*)
SI_UNIT(.CENTI.,.METRE.)
);
#9288=(
NAMED_UNIT(*)
PLANE_ANGLE_UNIT()
SI_UNIT($,.RADIAN.)
);
#9289=(
NAMED_UNIT(*)
SI_UNIT($,.STERADIAN.)
SOLID_ANGLE_UNIT()
);
#9292=SHAPE_DEFINITION_REPRESENTATION(#9321,#9396);
#9321=PRODUCT_DEFINITION_SHAPE('',$,#9426);
#9396=SHAPE_REPRESENTATION('',(#5463),#9258);
#9423=PRODUCT_DEFINITION_CONTEXT('part definition',#9512,'design');
#9426=PRODUCT_DEFINITION('Twenty-five millimetre clamp base',
'Twenty-five millimetre clamp base',#9455,#9423);
#9455=PRODUCT_DEFINITION_FORMATION('',$,#9516);
#9512=APPLICATION_CONTEXT(
'Core Data for Automotive Mechanical Design Process');
#9513=PRODUCT_CONTEXT('part definition',#9512,'mechanical');
#9516=PRODUCT('Twenty-five millimetre clamp base',
'Twenty-five millimetre clamp base','Twenty-five millimetre clamp base',
(#9513));
#9585=COLOUR_RGB('Dark Blue',0.08,0.2,0.34);
#9586=FILL_AREA_STYLE_COLOUR('',#9585);
#9587=FILL_AREA_STYLE('',(#9586));
#9588=SURFACE_STYLE_FILL_AREA(#9587);
#9589=SURFACE_SIDE_STYLE('',(#9588));
#9590=SURFACE_STYLE_USAGE(.BOTH.,#9589);
#9591=PRESENTATION_STYLE_ASSIGNMENT((#9590));
ENDSEC;
END-ISO-10303-21;
